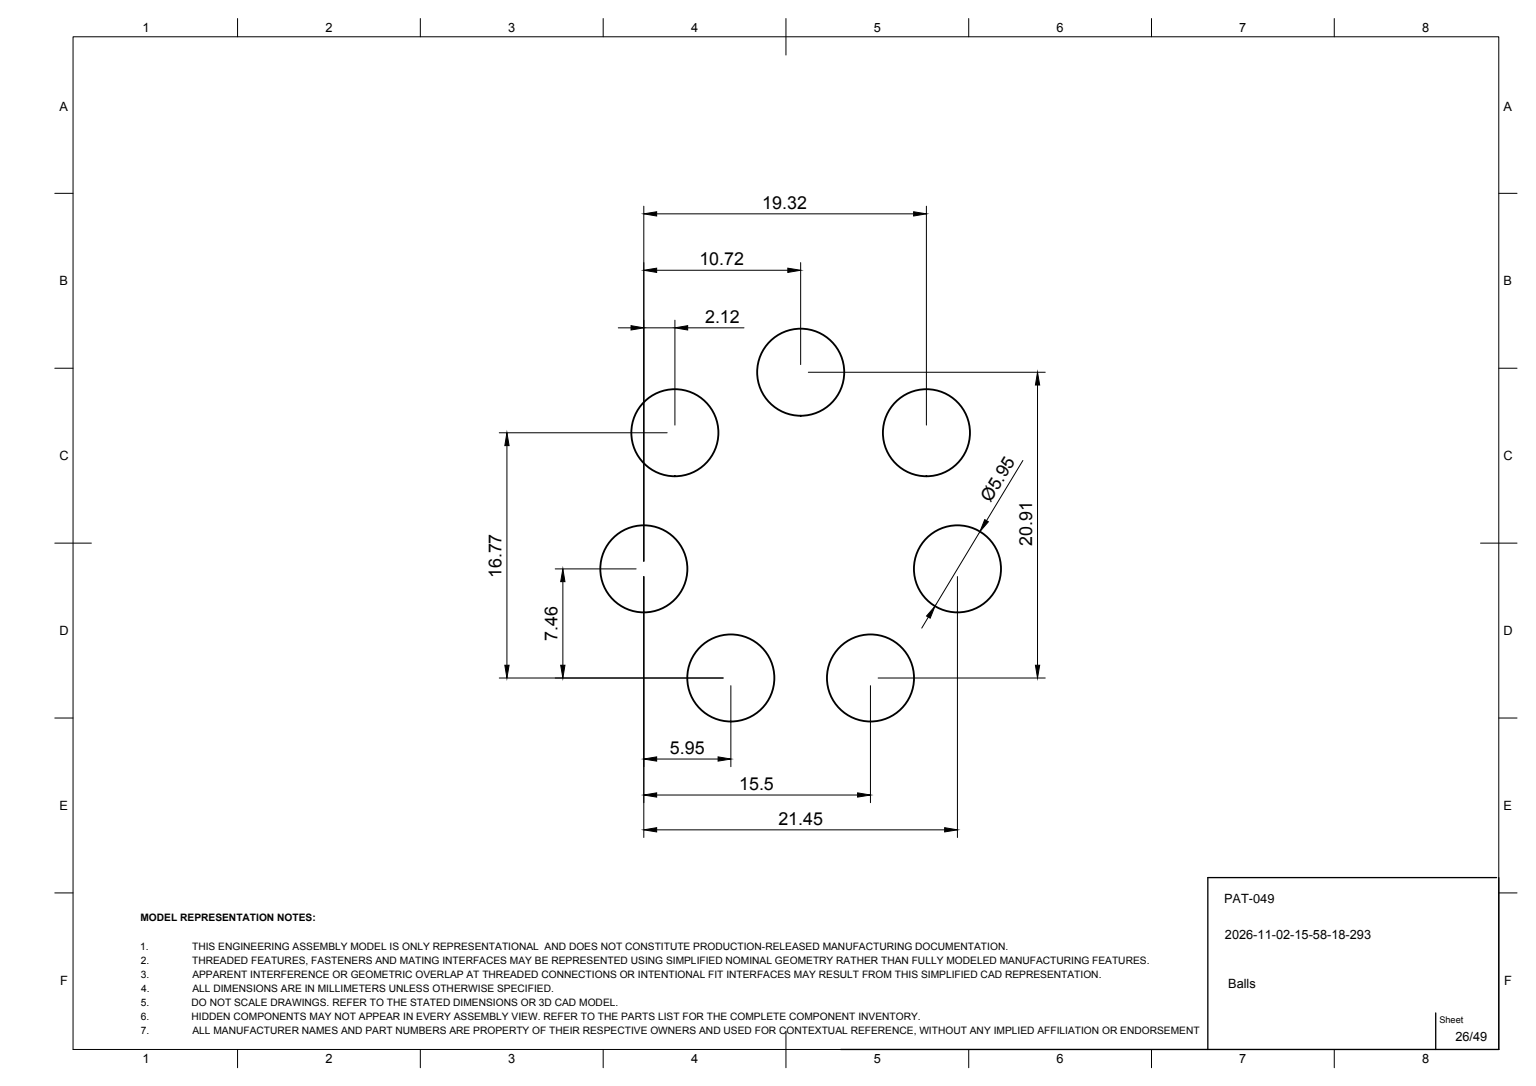
ISO-10303-21;
HEADER;
/* Generated by software containing ST-Developer
 * from STEP Tools, Inc. (www.steptools.com) 
 */

FILE_DESCRIPTION(
/* description */ ('Hand drill press frame (manual)'),
/* implementation_level */ '2;1');

FILE_NAME(
/* name */ 'Balls.step',
/* time_stamp */ '2026-10-28T03:25:28-07:00',
/* author */ (''),
/* organization */ (''),
/* preprocessor_version */ 'ST-DEVELOPER v20.2',
/* originating_system */ 'Autodesk Translation Framework v15.17.0.0',
/* authorisation */ '');

FILE_SCHEMA (('AUTOMOTIVE_DESIGN { 1 0 10303 214 3 1 1 }'));
ENDSEC;

DATA;
#10=MECHANICAL_DESIGN_GEOMETRIC_PRESENTATION_REPRESENTATION('',(#638,#639,#640,#641,#642,#643,#644),#33299);
#457=SPHERICAL_SURFACE('',#13645,0.29765);
#458=SPHERICAL_SURFACE('',#13647,0.29765);
#459=SPHERICAL_SURFACE('',#13649,0.29765);
#460=SPHERICAL_SURFACE('',#13651,0.29765);
#461=SPHERICAL_SURFACE('',#13653,0.29765);
#462=SPHERICAL_SURFACE('',#13655,0.29765);
#463=SPHERICAL_SURFACE('',#13657,0.29765);
#548=SHAPE_REPRESENTATION_RELATIONSHIP('SRR','None',#33508,#593);
#593=ADVANCED_BREP_SHAPE_REPRESENTATION('',(#690,#691,#692,#693,#694,#695,
#696),#33270);
#638=STYLED_ITEM('',(#33814),#690);
#639=STYLED_ITEM('',(#33814),#691);
#640=STYLED_ITEM('',(#33814),#692);
#641=STYLED_ITEM('',(#33814),#693);
#642=STYLED_ITEM('',(#33814),#694);
#643=STYLED_ITEM('',(#33814),#695);
#644=STYLED_ITEM('',(#33814),#696);
#690=MANIFOLD_SOLID_BREP('Body1',#12656);
#691=MANIFOLD_SOLID_BREP('Body2',#12657);
#692=MANIFOLD_SOLID_BREP('Body3',#12658);
#693=MANIFOLD_SOLID_BREP('Body4',#12659);
#694=MANIFOLD_SOLID_BREP('Body5',#12660);
#695=MANIFOLD_SOLID_BREP('Body6',#12661);
#696=MANIFOLD_SOLID_BREP('Body7',#12662);
#1572=FACE_OUTER_BOUND('',#2381,.T.);
#1573=FACE_OUTER_BOUND('',#2382,.T.);
#1574=FACE_OUTER_BOUND('',#2383,.T.);
#1575=FACE_OUTER_BOUND('',#2384,.T.);
#1576=FACE_OUTER_BOUND('',#2385,.T.);
#1577=FACE_OUTER_BOUND('',#2386,.T.);
#1578=FACE_OUTER_BOUND('',#2387,.T.);
#2381=EDGE_LOOP('',(#9511,#9512));
#2382=EDGE_LOOP('',(#9513,#9514));
#2383=EDGE_LOOP('',(#9515,#9516));
#2384=EDGE_LOOP('',(#9517,#9518));
#2385=EDGE_LOOP('',(#9519,#9520));
#2386=EDGE_LOOP('',(#9521,#9522));
#2387=EDGE_LOOP('',(#9523,#9524));
#5415=CIRCLE('',#13646,0.29765);
#5416=CIRCLE('',#13648,0.29765);
#5417=CIRCLE('',#13650,0.29765);
#5418=CIRCLE('',#13652,0.29765);
#5419=CIRCLE('',#13654,0.29765);
#5420=CIRCLE('',#13656,0.29765);
#5421=CIRCLE('',#13658,0.29765);
#5975=VERTEX_POINT('',#19237);
#5976=VERTEX_POINT('',#19238);
#5977=VERTEX_POINT('',#19241);
#5978=VERTEX_POINT('',#19242);
#5979=VERTEX_POINT('',#19245);
#5980=VERTEX_POINT('',#19246);
#5981=VERTEX_POINT('',#19249);
#5982=VERTEX_POINT('',#19250);
#5983=VERTEX_POINT('',#19253);
#5984=VERTEX_POINT('',#19254);
#5985=VERTEX_POINT('',#19257);
#5986=VERTEX_POINT('',#19258);
#5987=VERTEX_POINT('',#19261);
#5988=VERTEX_POINT('',#19262);
#7284=EDGE_CURVE('',#5975,#5976,#5415,.T.);
#7285=EDGE_CURVE('',#5977,#5978,#5416,.T.);
#7286=EDGE_CURVE('',#5979,#5980,#5417,.T.);
#7287=EDGE_CURVE('',#5981,#5982,#5418,.T.);
#7288=EDGE_CURVE('',#5983,#5984,#5419,.T.);
#7289=EDGE_CURVE('',#5985,#5986,#5420,.T.);
#7290=EDGE_CURVE('',#5987,#5988,#5421,.T.);
#9511=ORIENTED_EDGE('',*,*,#7284,.T.);
#9512=ORIENTED_EDGE('',*,*,#7284,.F.);
#9513=ORIENTED_EDGE('',*,*,#7285,.T.);
#9514=ORIENTED_EDGE('',*,*,#7285,.F.);
#9515=ORIENTED_EDGE('',*,*,#7286,.T.);
#9516=ORIENTED_EDGE('',*,*,#7286,.F.);
#9517=ORIENTED_EDGE('',*,*,#7287,.T.);
#9518=ORIENTED_EDGE('',*,*,#7287,.F.);
#9519=ORIENTED_EDGE('',*,*,#7288,.T.);
#9520=ORIENTED_EDGE('',*,*,#7288,.F.);
#9521=ORIENTED_EDGE('',*,*,#7289,.T.);
#9522=ORIENTED_EDGE('',*,*,#7289,.F.);
#9523=ORIENTED_EDGE('',*,*,#7290,.T.);
#9524=ORIENTED_EDGE('',*,*,#7290,.F.);
#12181=ADVANCED_FACE('',(#1572),#457,.T.);
#12182=ADVANCED_FACE('',(#1573),#458,.T.);
#12183=ADVANCED_FACE('',(#1574),#459,.T.);
#12184=ADVANCED_FACE('',(#1575),#460,.T.);
#12185=ADVANCED_FACE('',(#1576),#461,.T.);
#12186=ADVANCED_FACE('',(#1577),#462,.T.);
#12187=ADVANCED_FACE('',(#1578),#463,.T.);
#12656=CLOSED_SHELL('',(#12181));
#12657=CLOSED_SHELL('',(#12182));
#12658=CLOSED_SHELL('',(#12183));
#12659=CLOSED_SHELL('',(#12184));
#12660=CLOSED_SHELL('',(#12185));
#12661=CLOSED_SHELL('',(#12186));
#12662=CLOSED_SHELL('',(#12187));
#13644=AXIS2_PLACEMENT_3D('',#19235,#15608,#15609);
#13645=AXIS2_PLACEMENT_3D('',#19236,#15610,#15611);
#13646=AXIS2_PLACEMENT_3D('',#19239,#15612,#15613);
#13647=AXIS2_PLACEMENT_3D('',#19240,#15614,#15615);
#13648=AXIS2_PLACEMENT_3D('',#19243,#15616,#15617);
#13649=AXIS2_PLACEMENT_3D('',#19244,#15618,#15619);
#13650=AXIS2_PLACEMENT_3D('',#19247,#15620,#15621);
#13651=AXIS2_PLACEMENT_3D('',#19248,#15622,#15623);
#13652=AXIS2_PLACEMENT_3D('',#19251,#15624,#15625);
#13653=AXIS2_PLACEMENT_3D('',#19252,#15626,#15627);
#13654=AXIS2_PLACEMENT_3D('',#19255,#15628,#15629);
#13655=AXIS2_PLACEMENT_3D('',#19256,#15630,#15631);
#13656=AXIS2_PLACEMENT_3D('',#19259,#15632,#15633);
#13657=AXIS2_PLACEMENT_3D('',#19260,#15634,#15635);
#13658=AXIS2_PLACEMENT_3D('',#19263,#15636,#15637);
#15608=DIRECTION('axis',(0.,0.,1.));
#15609=DIRECTION('refdir',(1.,0.,0.));
#15610=DIRECTION('center_axis',(0.,0.,1.));
#15611=DIRECTION('ref_axis',(1.,0.,0.));
#15612=DIRECTION('center_axis',(1.22464679914735E-16,-1.,0.));
#15613=DIRECTION('ref_axis',(-1.,-1.22464679914735E-16,0.));
#15614=DIRECTION('center_axis',(0.78183148246803,0.,0.623489801858733));
#15615=DIRECTION('ref_axis',(0.623489801858734,0.,-0.78183148246803));
#15616=DIRECTION('center_axis',(7.63554790147315E-17,-1.,-9.57467422477103E-17));
#15617=DIRECTION('ref_axis',(-0.623489801858734,-1.22464679914735E-16,0.78183148246803));
#15618=DIRECTION('center_axis',(0.974927912181824,0.,-0.222520933956314));
#15619=DIRECTION('ref_axis',(-0.222520933956314,0.,-0.974927912181824));
#15620=DIRECTION('center_axis',(-2.7250954951288E-17,-1.,-1.19394234705288E-16));
#15621=DIRECTION('ref_axis',(0.222520933956314,-1.22464679914735E-16,0.974927912181824));
#15622=DIRECTION('center_axis',(0.433883739117558,0.,-0.900968867902419));
#15623=DIRECTION('ref_axis',(-0.900968867902419,0.,-0.433883739117558));
#15624=DIRECTION('center_axis',(-1.10336864020811E-16,-1.,-5.31354332312403E-17));
#15625=DIRECTION('ref_axis',(0.900968867902419,-1.22464679914735E-16,0.433883739117558));
#15626=DIRECTION('center_axis',(-0.433883739117558,0.,-0.900968867902419));
#15627=DIRECTION('ref_axis',(-0.900968867902419,0.,0.433883739117558));
#15628=DIRECTION('center_axis',(-1.10336864020811E-16,-1.,5.31354332312403E-17));
#15629=DIRECTION('ref_axis',(0.900968867902419,-1.22464679914735E-16,-0.433883739117558));
#15630=DIRECTION('center_axis',(-0.974927912181824,0.,-0.222520933956314));
#15631=DIRECTION('ref_axis',(-0.222520933956315,0.,0.974927912181824));
#15632=DIRECTION('center_axis',(-2.7250954951288E-17,-1.,1.19394234705288E-16));
#15633=DIRECTION('ref_axis',(0.222520933956315,-1.22464679914735E-16,-0.974927912181824));
#15634=DIRECTION('center_axis',(-0.78183148246803,0.,0.623489801858734));
#15635=DIRECTION('ref_axis',(0.623489801858733,0.,0.78183148246803));
#15636=DIRECTION('center_axis',(7.63554790147315E-17,-1.,9.57467422477103E-17));
#15637=DIRECTION('ref_axis',(-0.623489801858733,-1.22464679914735E-16,-0.78183148246803));
#19235=CARTESIAN_POINT('',(0.,0.,0.));
#19236=CARTESIAN_POINT('Origin',(1.1,0.,0.));
#19237=CARTESIAN_POINT('',(1.1,-2.23201749654651E-33,0.29765));
#19238=CARTESIAN_POINT('',(1.1,-2.23201749654651E-33,-0.29765));
#19239=CARTESIAN_POINT('Origin',(1.1,0.,0.));
#19240=CARTESIAN_POINT('Origin',(0.685838782044607,0.,-0.860014630714833));
#19241=CARTESIAN_POINT('',(0.918550922801216,-5.31350540756609E-33,-0.674432891191581));
#19242=CARTESIAN_POINT('',(0.453126641287998,8.49470414473068E-34,-1.04559637023808));
#19243=CARTESIAN_POINT('Origin',(0.685838782044607,0.,-0.860014630714833));
#19244=CARTESIAN_POINT('Origin',(-0.244773027351946,0.,-1.07242070340001));
#19245=CARTESIAN_POINT('',(0.0454142657089739,-2.23201749654651E-33,-1.1386540593921));
#19246=CARTESIAN_POINT('',(-0.534960320412865,-2.23201749654651E-33,-1.00618734740791));
#19247=CARTESIAN_POINT('Origin',(-0.244773027351946,0.,-1.07242070340001));
#19248=CARTESIAN_POINT('Origin',(-0.991065754692661,0.,-0.477272113029314));
#19249=CARTESIAN_POINT('',(-0.86192025974432,8.49470414473067E-34,-0.745445496560469));
#19250=CARTESIAN_POINT('',(-1.120211249641,-5.31350540756609E-33,-0.209098729498159));
#19251=CARTESIAN_POINT('Origin',(-0.991065754692661,0.,-0.477272113029314));
#19252=CARTESIAN_POINT('Origin',(-0.991065754692661,0.,0.477272113029314));
#19253=CARTESIAN_POINT('',(-1.120211249641,-2.23201749654651E-33,0.209098729498159));
#19254=CARTESIAN_POINT('',(-0.86192025974432,-2.23201749654651E-33,0.745445496560469));
#19255=CARTESIAN_POINT('Origin',(-0.991065754692661,0.,0.477272113029314));
#19256=CARTESIAN_POINT('Origin',(-0.244773027351946,0.,1.07242070340001));
#19257=CARTESIAN_POINT('',(-0.534960320412866,-2.23201749654651E-33,1.00618734740791));
#19258=CARTESIAN_POINT('',(0.0454142657089737,-2.23201749654651E-33,1.1386540593921));
#19259=CARTESIAN_POINT('Origin',(-0.244773027351946,0.,1.07242070340001));
#19260=CARTESIAN_POINT('Origin',(0.685838782044607,0.,0.860014630714833));
#19261=CARTESIAN_POINT('',(0.453126641287998,-2.23201749654651E-33,1.04559637023808));
#19262=CARTESIAN_POINT('',(0.918550922801216,-2.23201749654651E-33,0.674432891191581));
#19263=CARTESIAN_POINT('Origin',(0.685838782044607,0.,0.860014630714833));
#33218=UNCERTAINTY_MEASURE_WITH_UNIT(LENGTH_MEASURE(0.001),#33300,
'DISTANCE_ACCURACY_VALUE',
'Maximum model space distance between geometric entities at asserted c
onnectivities');
#33247=UNCERTAINTY_MEASURE_WITH_UNIT(LENGTH_MEASURE(0.001),#33300,
'DISTANCE_ACCURACY_VALUE',
'Maximum model space distance between geometric entities at asserted c
onnectivities');
#33270=(
GEOMETRIC_REPRESENTATION_CONTEXT(3)
GLOBAL_UNCERTAINTY_ASSIGNED_CONTEXT((#33218))
GLOBAL_UNIT_ASSIGNED_CONTEXT((#33300,#33302,#33303))
REPRESENTATION_CONTEXT('','3D')
);
#33299=(
GEOMETRIC_REPRESENTATION_CONTEXT(3)
GLOBAL_UNCERTAINTY_ASSIGNED_CONTEXT((#33247))
GLOBAL_UNIT_ASSIGNED_CONTEXT((#33300,#33302,#33303))
REPRESENTATION_CONTEXT('','3D')
);
#33300=(
LENGTH_UNIT()
NAMED_UNIT(*)
SI_UNIT(.CENTI.,.METRE.)
);
#33302=(
NAMED_UNIT(*)
PLANE_ANGLE_UNIT()
SI_UNIT($,.RADIAN.)
);
#33303=(
NAMED_UNIT(*)
SI_UNIT($,.STERADIAN.)
SOLID_ANGLE_UNIT()
);
#33326=SHAPE_DEFINITION_REPRESENTATION(#33377,#33508);
#33377=PRODUCT_DEFINITION_SHAPE('',$,#33560);
#33508=SHAPE_REPRESENTATION('',(#13644),#33270);
#33537=PRODUCT_DEFINITION_CONTEXT('part definition',#33692,'design');
#33560=PRODUCT_DEFINITION('Balls','Balls',#33611,#33537);
#33611=PRODUCT_DEFINITION_FORMATION('',$,#33716);
#33692=APPLICATION_CONTEXT(
'Core Data for Automotive Mechanical Design Process');
#33693=PRODUCT_CONTEXT('part definition',#33692,'mechanical');
#33716=PRODUCT('Balls','Balls','Balls',(#33693));
#33808=COLOUR_RGB('Grey',0.48,0.52,0.57);
#33809=FILL_AREA_STYLE_COLOUR('',#33808);
#33810=FILL_AREA_STYLE('',(#33809));
#33811=SURFACE_STYLE_FILL_AREA(#33810);
#33812=SURFACE_SIDE_STYLE('',(#33811));
#33813=SURFACE_STYLE_USAGE(.BOTH.,#33812);
#33814=PRESENTATION_STYLE_ASSIGNMENT((#33813));
ENDSEC;
END-ISO-10303-21;
